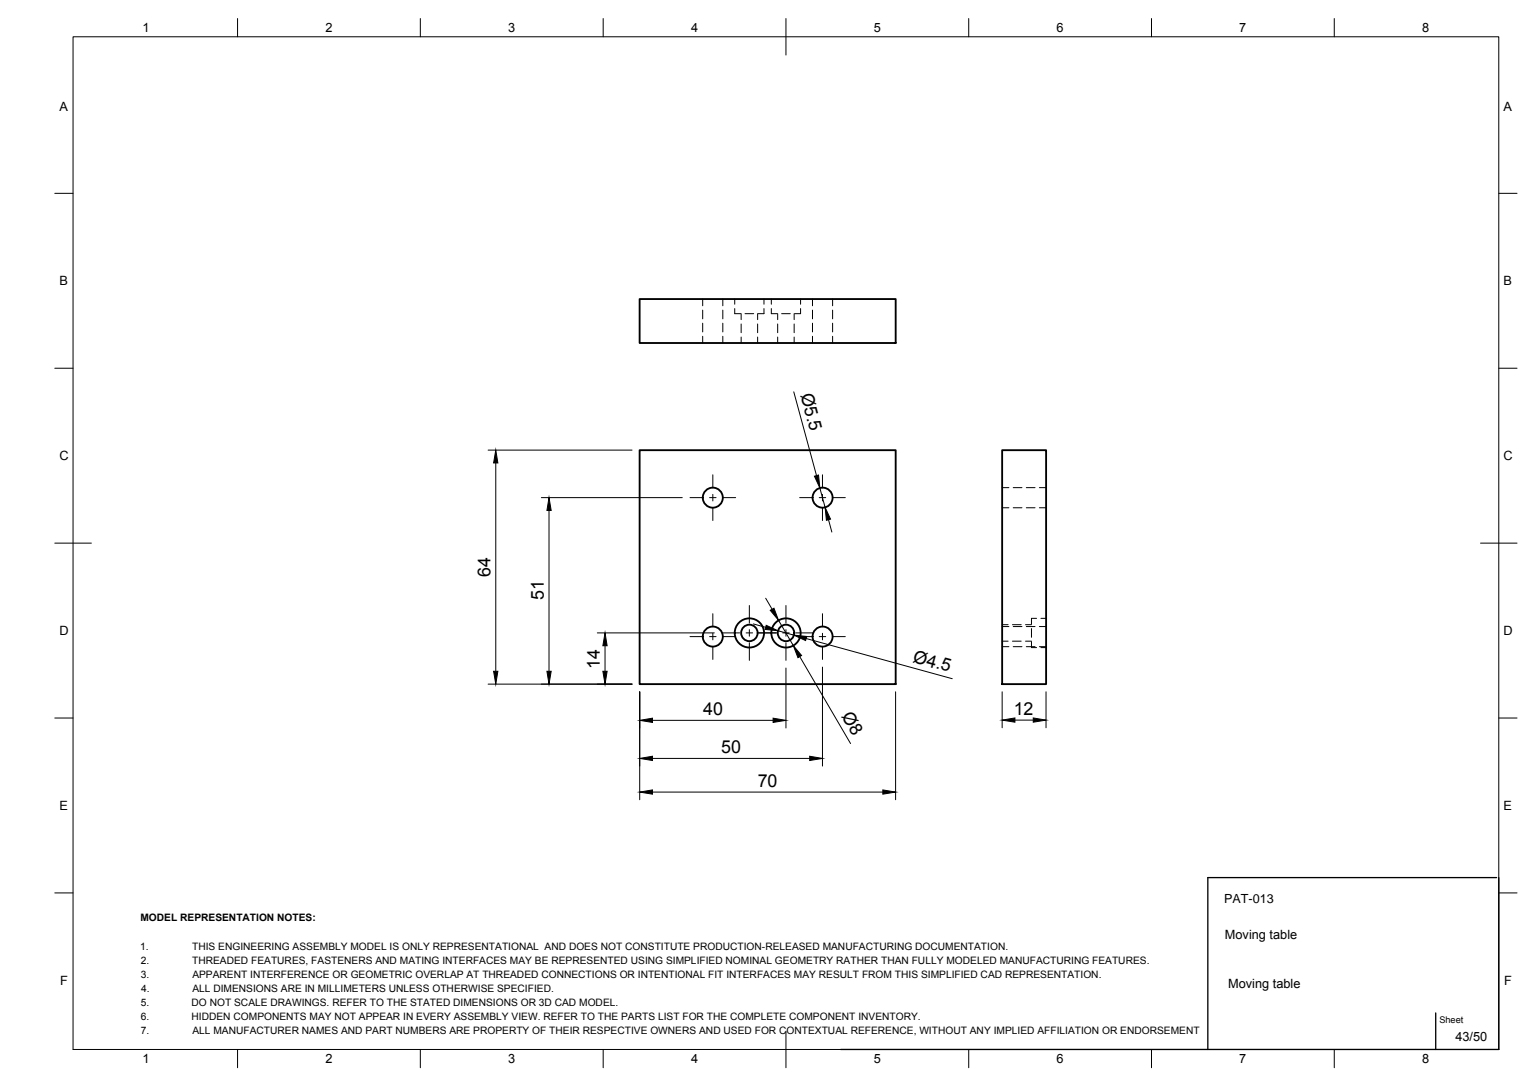
ISO-10303-21;
HEADER;
/* Generated by software containing ST-Developer
 * from STEP Tools, Inc. (www.steptools.com) 
 */

FILE_DESCRIPTION(
/* description */ ('Belt-driven linear axis on 2020 extrusion'),
/* implementation_level */ '2;1');

FILE_NAME(
/* name */ 'Moving table.step',
/* time_stamp */ '2026-10-28T03:26:09-07:00',
/* author */ (''),
/* organization */ (''),
/* preprocessor_version */ 'ST-DEVELOPER v20.2',
/* originating_system */ 'Autodesk Translation Framework v15.17.0.0',
/* authorisation */ '');

FILE_SCHEMA (('AUTOMOTIVE_DESIGN { 1 0 10303 214 3 1 1 }'));
ENDSEC;

DATA;
#10=MECHANICAL_DESIGN_GEOMETRIC_PRESENTATION_REPRESENTATION('',(#656),#20096);
#554=SHAPE_REPRESENTATION_RELATIONSHIP('SRR','None',#20354,#600);
#600=ADVANCED_BREP_SHAPE_REPRESENTATION('',(#711),#20085);
#656=STYLED_ITEM('',(#20643),#711);
#711=MANIFOLD_SOLID_BREP('Body1',#10970);
#862=FACE_BOUND('',#2501,.T.);
#863=FACE_BOUND('',#2504,.T.);
#864=FACE_BOUND('',#2516,.T.);
#865=FACE_BOUND('',#2517,.T.);
#866=FACE_BOUND('',#2518,.T.);
#867=FACE_BOUND('',#2519,.T.);
#868=FACE_BOUND('',#2520,.T.);
#869=FACE_BOUND('',#2521,.T.);
#870=FACE_BOUND('',#2523,.T.);
#871=FACE_BOUND('',#2524,.T.);
#872=FACE_BOUND('',#2525,.T.);
#873=FACE_BOUND('',#2526,.T.);
#874=FACE_BOUND('',#2527,.T.);
#875=FACE_BOUND('',#2528,.T.);
#1149=PLANE('',#12467);
#1150=PLANE('',#12472);
#1151=PLANE('',#12490);
#1152=PLANE('',#12491);
#1153=PLANE('',#12492);
#1154=PLANE('',#12493);
#1155=PLANE('',#12494);
#1156=PLANE('',#12495);
#1733=FACE_OUTER_BOUND('',#2499,.T.);
#1734=FACE_OUTER_BOUND('',#2500,.T.);
#1735=FACE_OUTER_BOUND('',#2502,.T.);
#1736=FACE_OUTER_BOUND('',#2503,.T.);
#1737=FACE_OUTER_BOUND('',#2505,.T.);
#1738=FACE_OUTER_BOUND('',#2506,.T.);
#1739=FACE_OUTER_BOUND('',#2507,.T.);
#1740=FACE_OUTER_BOUND('',#2508,.T.);
#1741=FACE_OUTER_BOUND('',#2509,.T.);
#1742=FACE_OUTER_BOUND('',#2510,.T.);
#1743=FACE_OUTER_BOUND('',#2511,.T.);
#1744=FACE_OUTER_BOUND('',#2512,.T.);
#1745=FACE_OUTER_BOUND('',#2513,.T.);
#1746=FACE_OUTER_BOUND('',#2514,.T.);
#1747=FACE_OUTER_BOUND('',#2515,.T.);
#1748=FACE_OUTER_BOUND('',#2522,.T.);
#2499=EDGE_LOOP('',(#9453,#9454,#9455,#9456));
#2500=EDGE_LOOP('',(#9457));
#2501=EDGE_LOOP('',(#9458));
#2502=EDGE_LOOP('',(#9459,#9460,#9461,#9462));
#2503=EDGE_LOOP('',(#9463));
#2504=EDGE_LOOP('',(#9464));
#2505=EDGE_LOOP('',(#9465,#9466,#9467,#9468));
#2506=EDGE_LOOP('',(#9469,#9470,#9471,#9472));
#2507=EDGE_LOOP('',(#9473,#9474,#9475,#9476));
#2508=EDGE_LOOP('',(#9477,#9478,#9479,#9480));
#2509=EDGE_LOOP('',(#9481,#9482,#9483,#9484));
#2510=EDGE_LOOP('',(#9485,#9486,#9487,#9488));
#2511=EDGE_LOOP('',(#9489,#9490,#9491,#9492));
#2512=EDGE_LOOP('',(#9493,#9494,#9495,#9496));
#2513=EDGE_LOOP('',(#9497,#9498,#9499,#9500));
#2514=EDGE_LOOP('',(#9501,#9502,#9503,#9504));
#2515=EDGE_LOOP('',(#9505,#9506,#9507,#9508));
#2516=EDGE_LOOP('',(#9509));
#2517=EDGE_LOOP('',(#9510));
#2518=EDGE_LOOP('',(#9511));
#2519=EDGE_LOOP('',(#9512));
#2520=EDGE_LOOP('',(#9513));
#2521=EDGE_LOOP('',(#9514));
#2522=EDGE_LOOP('',(#9515,#9516,#9517,#9518));
#2523=EDGE_LOOP('',(#9519));
#2524=EDGE_LOOP('',(#9520));
#2525=EDGE_LOOP('',(#9521));
#2526=EDGE_LOOP('',(#9522));
#2527=EDGE_LOOP('',(#9523));
#2528=EDGE_LOOP('',(#9524));
#3282=LINE('',#19228,#4139);
#3283=LINE('',#19237,#4140);
#3284=LINE('',#19244,#4141);
#3285=LINE('',#19248,#4142);
#3286=LINE('',#19254,#4143);
#3287=LINE('',#19260,#4144);
#3288=LINE('',#19266,#4145);
#3289=LINE('',#19272,#4146);
#3290=LINE('',#19277,#4147);
#3291=LINE('',#19279,#4148);
#3292=LINE('',#19281,#4149);
#3293=LINE('',#19282,#4150);
#3294=LINE('',#19285,#4151);
#3295=LINE('',#19287,#4152);
#3296=LINE('',#19288,#4153);
#3297=LINE('',#19291,#4154);
#3298=LINE('',#19293,#4155);
#3299=LINE('',#19294,#4156);
#3300=LINE('',#19296,#4157);
#3301=LINE('',#19297,#4158);
#4139=VECTOR('',#15354,0.4);
#4140=VECTOR('',#15365,0.399999999999999);
#4141=VECTOR('',#15374,0.225);
#4142=VECTOR('',#15379,0.225000000000001);
#4143=VECTOR('',#15386,0.274999999999999);
#4144=VECTOR('',#15393,0.275);
#4145=VECTOR('',#15400,0.275);
#4146=VECTOR('',#15407,0.274999999999999);
#4147=VECTOR('',#15412,1.);
#4148=VECTOR('',#15413,1.);
#4149=VECTOR('',#15414,1.);
#4150=VECTOR('',#15415,1.);
#4151=VECTOR('',#15418,1.);
#4152=VECTOR('',#15419,1.);
#4153=VECTOR('',#15420,1.);
#4154=VECTOR('',#15423,1.);
#4155=VECTOR('',#15424,1.);
#4156=VECTOR('',#15425,1.);
#4157=VECTOR('',#15428,1.);
#4158=VECTOR('',#15429,1.);
#4820=CIRCLE('',#12465,0.4);
#4821=CIRCLE('',#12466,0.4);
#4822=CIRCLE('',#12468,0.225);
#4823=CIRCLE('',#12470,0.399999999999999);
#4824=CIRCLE('',#12471,0.399999999999999);
#4825=CIRCLE('',#12473,0.225000000000001);
#4826=CIRCLE('',#12475,0.225);
#4827=CIRCLE('',#12477,0.225000000000001);
#4828=CIRCLE('',#12479,0.274999999999999);
#4829=CIRCLE('',#12480,0.274999999999999);
#4830=CIRCLE('',#12482,0.275);
#4831=CIRCLE('',#12483,0.275);
#4832=CIRCLE('',#12485,0.275);
#4833=CIRCLE('',#12486,0.275);
#4834=CIRCLE('',#12488,0.274999999999999);
#4835=CIRCLE('',#12489,0.274999999999999);
#5637=VERTEX_POINT('',#19225);
#5638=VERTEX_POINT('',#19227);
#5639=VERTEX_POINT('',#19231);
#5640=VERTEX_POINT('',#19234);
#5641=VERTEX_POINT('',#19236);
#5642=VERTEX_POINT('',#19240);
#5643=VERTEX_POINT('',#19243);
#5644=VERTEX_POINT('',#19247);
#5645=VERTEX_POINT('',#19251);
#5646=VERTEX_POINT('',#19253);
#5647=VERTEX_POINT('',#19257);
#5648=VERTEX_POINT('',#19259);
#5649=VERTEX_POINT('',#19263);
#5650=VERTEX_POINT('',#19265);
#5651=VERTEX_POINT('',#19269);
#5652=VERTEX_POINT('',#19271);
#5653=VERTEX_POINT('',#19275);
#5654=VERTEX_POINT('',#19276);
#5655=VERTEX_POINT('',#19278);
#5656=VERTEX_POINT('',#19280);
#5657=VERTEX_POINT('',#19284);
#5658=VERTEX_POINT('',#19286);
#5659=VERTEX_POINT('',#19290);
#5660=VERTEX_POINT('',#19292);
#6941=EDGE_CURVE('',#5637,#5637,#4820,.T.);
#6942=EDGE_CURVE('',#5637,#5638,#3282,.T.);
#6943=EDGE_CURVE('',#5638,#5638,#4821,.T.);
#6944=EDGE_CURVE('',#5639,#5639,#4822,.T.);
#6945=EDGE_CURVE('',#5640,#5640,#4823,.T.);
#6946=EDGE_CURVE('',#5640,#5641,#3283,.T.);
#6947=EDGE_CURVE('',#5641,#5641,#4824,.T.);
#6948=EDGE_CURVE('',#5642,#5642,#4825,.T.);
#6949=EDGE_CURVE('',#5639,#5643,#3284,.T.);
#6950=EDGE_CURVE('',#5643,#5643,#4826,.T.);
#6951=EDGE_CURVE('',#5642,#5644,#3285,.T.);
#6952=EDGE_CURVE('',#5644,#5644,#4827,.T.);
#6953=EDGE_CURVE('',#5645,#5645,#4828,.T.);
#6954=EDGE_CURVE('',#5645,#5646,#3286,.T.);
#6955=EDGE_CURVE('',#5646,#5646,#4829,.T.);
#6956=EDGE_CURVE('',#5647,#5647,#4830,.T.);
#6957=EDGE_CURVE('',#5647,#5648,#3287,.T.);
#6958=EDGE_CURVE('',#5648,#5648,#4831,.T.);
#6959=EDGE_CURVE('',#5649,#5649,#4832,.T.);
#6960=EDGE_CURVE('',#5649,#5650,#3288,.T.);
#6961=EDGE_CURVE('',#5650,#5650,#4833,.T.);
#6962=EDGE_CURVE('',#5651,#5651,#4834,.T.);
#6963=EDGE_CURVE('',#5651,#5652,#3289,.T.);
#6964=EDGE_CURVE('',#5652,#5652,#4835,.T.);
#6965=EDGE_CURVE('',#5653,#5654,#3290,.T.);
#6966=EDGE_CURVE('',#5654,#5655,#3291,.T.);
#6967=EDGE_CURVE('',#5656,#5655,#3292,.T.);
#6968=EDGE_CURVE('',#5653,#5656,#3293,.T.);
#6969=EDGE_CURVE('',#5657,#5653,#3294,.T.);
#6970=EDGE_CURVE('',#5658,#5656,#3295,.T.);
#6971=EDGE_CURVE('',#5657,#5658,#3296,.T.);
#6972=EDGE_CURVE('',#5659,#5657,#3297,.T.);
#6973=EDGE_CURVE('',#5660,#5658,#3298,.T.);
#6974=EDGE_CURVE('',#5659,#5660,#3299,.T.);
#6975=EDGE_CURVE('',#5654,#5659,#3300,.T.);
#6976=EDGE_CURVE('',#5655,#5660,#3301,.T.);
#9453=ORIENTED_EDGE('',*,*,#6941,.F.);
#9454=ORIENTED_EDGE('',*,*,#6942,.T.);
#9455=ORIENTED_EDGE('',*,*,#6943,.T.);
#9456=ORIENTED_EDGE('',*,*,#6942,.F.);
#9457=ORIENTED_EDGE('',*,*,#6943,.F.);
#9458=ORIENTED_EDGE('',*,*,#6944,.F.);
#9459=ORIENTED_EDGE('',*,*,#6945,.F.);
#9460=ORIENTED_EDGE('',*,*,#6946,.T.);
#9461=ORIENTED_EDGE('',*,*,#6947,.T.);
#9462=ORIENTED_EDGE('',*,*,#6946,.F.);
#9463=ORIENTED_EDGE('',*,*,#6947,.F.);
#9464=ORIENTED_EDGE('',*,*,#6948,.F.);
#9465=ORIENTED_EDGE('',*,*,#6944,.T.);
#9466=ORIENTED_EDGE('',*,*,#6949,.T.);
#9467=ORIENTED_EDGE('',*,*,#6950,.F.);
#9468=ORIENTED_EDGE('',*,*,#6949,.F.);
#9469=ORIENTED_EDGE('',*,*,#6948,.T.);
#9470=ORIENTED_EDGE('',*,*,#6951,.T.);
#9471=ORIENTED_EDGE('',*,*,#6952,.F.);
#9472=ORIENTED_EDGE('',*,*,#6951,.F.);
#9473=ORIENTED_EDGE('',*,*,#6953,.F.);
#9474=ORIENTED_EDGE('',*,*,#6954,.T.);
#9475=ORIENTED_EDGE('',*,*,#6955,.F.);
#9476=ORIENTED_EDGE('',*,*,#6954,.F.);
#9477=ORIENTED_EDGE('',*,*,#6956,.F.);
#9478=ORIENTED_EDGE('',*,*,#6957,.T.);
#9479=ORIENTED_EDGE('',*,*,#6958,.F.);
#9480=ORIENTED_EDGE('',*,*,#6957,.F.);
#9481=ORIENTED_EDGE('',*,*,#6959,.F.);
#9482=ORIENTED_EDGE('',*,*,#6960,.T.);
#9483=ORIENTED_EDGE('',*,*,#6961,.F.);
#9484=ORIENTED_EDGE('',*,*,#6960,.F.);
#9485=ORIENTED_EDGE('',*,*,#6962,.F.);
#9486=ORIENTED_EDGE('',*,*,#6963,.T.);
#9487=ORIENTED_EDGE('',*,*,#6964,.F.);
#9488=ORIENTED_EDGE('',*,*,#6963,.F.);
#9489=ORIENTED_EDGE('',*,*,#6965,.T.);
#9490=ORIENTED_EDGE('',*,*,#6966,.T.);
#9491=ORIENTED_EDGE('',*,*,#6967,.F.);
#9492=ORIENTED_EDGE('',*,*,#6968,.F.);
#9493=ORIENTED_EDGE('',*,*,#6969,.T.);
#9494=ORIENTED_EDGE('',*,*,#6968,.T.);
#9495=ORIENTED_EDGE('',*,*,#6970,.F.);
#9496=ORIENTED_EDGE('',*,*,#6971,.F.);
#9497=ORIENTED_EDGE('',*,*,#6972,.T.);
#9498=ORIENTED_EDGE('',*,*,#6971,.T.);
#9499=ORIENTED_EDGE('',*,*,#6973,.F.);
#9500=ORIENTED_EDGE('',*,*,#6974,.F.);
#9501=ORIENTED_EDGE('',*,*,#6975,.T.);
#9502=ORIENTED_EDGE('',*,*,#6974,.T.);
#9503=ORIENTED_EDGE('',*,*,#6976,.F.);
#9504=ORIENTED_EDGE('',*,*,#6966,.F.);
#9505=ORIENTED_EDGE('',*,*,#6976,.T.);
#9506=ORIENTED_EDGE('',*,*,#6973,.T.);
#9507=ORIENTED_EDGE('',*,*,#6970,.T.);
#9508=ORIENTED_EDGE('',*,*,#6967,.T.);
#9509=ORIENTED_EDGE('',*,*,#6950,.T.);
#9510=ORIENTED_EDGE('',*,*,#6952,.T.);
#9511=ORIENTED_EDGE('',*,*,#6955,.T.);
#9512=ORIENTED_EDGE('',*,*,#6958,.T.);
#9513=ORIENTED_EDGE('',*,*,#6961,.T.);
#9514=ORIENTED_EDGE('',*,*,#6964,.T.);
#9515=ORIENTED_EDGE('',*,*,#6975,.F.);
#9516=ORIENTED_EDGE('',*,*,#6965,.F.);
#9517=ORIENTED_EDGE('',*,*,#6969,.F.);
#9518=ORIENTED_EDGE('',*,*,#6972,.F.);
#9519=ORIENTED_EDGE('',*,*,#6962,.T.);
#9520=ORIENTED_EDGE('',*,*,#6959,.T.);
#9521=ORIENTED_EDGE('',*,*,#6956,.T.);
#9522=ORIENTED_EDGE('',*,*,#6953,.T.);
#9523=ORIENTED_EDGE('',*,*,#6945,.T.);
#9524=ORIENTED_EDGE('',*,*,#6941,.T.);
#10275=CYLINDRICAL_SURFACE('',#12464,0.4);
#10276=CYLINDRICAL_SURFACE('',#12469,0.399999999999999);
#10277=CYLINDRICAL_SURFACE('',#12474,0.225);
#10278=CYLINDRICAL_SURFACE('',#12476,0.225000000000001);
#10279=CYLINDRICAL_SURFACE('',#12478,0.274999999999999);
#10280=CYLINDRICAL_SURFACE('',#12481,0.275);
#10281=CYLINDRICAL_SURFACE('',#12484,0.275);
#10282=CYLINDRICAL_SURFACE('',#12487,0.274999999999999);
#10784=ADVANCED_FACE('',(#1733),#10275,.F.);
#10785=ADVANCED_FACE('',(#1734,#862),#1149,.F.);
#10786=ADVANCED_FACE('',(#1735),#10276,.F.);
#10787=ADVANCED_FACE('',(#1736,#863),#1150,.F.);
#10788=ADVANCED_FACE('',(#1737),#10277,.F.);
#10789=ADVANCED_FACE('',(#1738),#10278,.F.);
#10790=ADVANCED_FACE('',(#1739),#10279,.F.);
#10791=ADVANCED_FACE('',(#1740),#10280,.F.);
#10792=ADVANCED_FACE('',(#1741),#10281,.F.);
#10793=ADVANCED_FACE('',(#1742),#10282,.F.);
#10794=ADVANCED_FACE('',(#1743),#1151,.T.);
#10795=ADVANCED_FACE('',(#1744),#1152,.T.);
#10796=ADVANCED_FACE('',(#1745),#1153,.T.);
#10797=ADVANCED_FACE('',(#1746),#1154,.T.);
#10798=ADVANCED_FACE('',(#1747,#864,#865,#866,#867,#868,#869),#1155,.T.);
#10799=ADVANCED_FACE('',(#1748,#870,#871,#872,#873,#874,#875),#1156,.F.);
#10970=CLOSED_SHELL('',(#10784,#10785,#10786,#10787,#10788,#10789,#10790,
#10791,#10792,#10793,#10794,#10795,#10796,#10797,#10798,#10799));
#12463=AXIS2_PLACEMENT_3D('',#19223,#15348,#15349);
#12464=AXIS2_PLACEMENT_3D('',#19224,#15350,#15351);
#12465=AXIS2_PLACEMENT_3D('',#19226,#15352,#15353);
#12466=AXIS2_PLACEMENT_3D('',#19229,#15355,#15356);
#12467=AXIS2_PLACEMENT_3D('',#19230,#15357,#15358);
#12468=AXIS2_PLACEMENT_3D('',#19232,#15359,#15360);
#12469=AXIS2_PLACEMENT_3D('',#19233,#15361,#15362);
#12470=AXIS2_PLACEMENT_3D('',#19235,#15363,#15364);
#12471=AXIS2_PLACEMENT_3D('',#19238,#15366,#15367);
#12472=AXIS2_PLACEMENT_3D('',#19239,#15368,#15369);
#12473=AXIS2_PLACEMENT_3D('',#19241,#15370,#15371);
#12474=AXIS2_PLACEMENT_3D('',#19242,#15372,#15373);
#12475=AXIS2_PLACEMENT_3D('',#19245,#15375,#15376);
#12476=AXIS2_PLACEMENT_3D('',#19246,#15377,#15378);
#12477=AXIS2_PLACEMENT_3D('',#19249,#15380,#15381);
#12478=AXIS2_PLACEMENT_3D('',#19250,#15382,#15383);
#12479=AXIS2_PLACEMENT_3D('',#19252,#15384,#15385);
#12480=AXIS2_PLACEMENT_3D('',#19255,#15387,#15388);
#12481=AXIS2_PLACEMENT_3D('',#19256,#15389,#15390);
#12482=AXIS2_PLACEMENT_3D('',#19258,#15391,#15392);
#12483=AXIS2_PLACEMENT_3D('',#19261,#15394,#15395);
#12484=AXIS2_PLACEMENT_3D('',#19262,#15396,#15397);
#12485=AXIS2_PLACEMENT_3D('',#19264,#15398,#15399);
#12486=AXIS2_PLACEMENT_3D('',#19267,#15401,#15402);
#12487=AXIS2_PLACEMENT_3D('',#19268,#15403,#15404);
#12488=AXIS2_PLACEMENT_3D('',#19270,#15405,#15406);
#12489=AXIS2_PLACEMENT_3D('',#19273,#15408,#15409);
#12490=AXIS2_PLACEMENT_3D('',#19274,#15410,#15411);
#12491=AXIS2_PLACEMENT_3D('',#19283,#15416,#15417);
#12492=AXIS2_PLACEMENT_3D('',#19289,#15421,#15422);
#12493=AXIS2_PLACEMENT_3D('',#19295,#15426,#15427);
#12494=AXIS2_PLACEMENT_3D('',#19298,#15430,#15431);
#12495=AXIS2_PLACEMENT_3D('',#19299,#15432,#15433);
#15348=DIRECTION('axis',(0.,0.,1.));
#15349=DIRECTION('refdir',(1.,0.,0.));
#15350=DIRECTION('center_axis',(0.,0.,1.));
#15351=DIRECTION('ref_axis',(1.,0.,0.));
#15352=DIRECTION('center_axis',(0.,0.,1.));
#15353=DIRECTION('ref_axis',(1.,0.,0.));
#15354=DIRECTION('',(0.,0.,1.));
#15355=DIRECTION('center_axis',(0.,0.,1.));
#15356=DIRECTION('ref_axis',(1.,0.,0.));
#15357=DIRECTION('center_axis',(0.,0.,1.));
#15358=DIRECTION('ref_axis',(1.,0.,0.));
#15359=DIRECTION('center_axis',(0.,0.,-1.));
#15360=DIRECTION('ref_axis',(1.,0.,0.));
#15361=DIRECTION('center_axis',(0.,0.,1.));
#15362=DIRECTION('ref_axis',(1.,0.,0.));
#15363=DIRECTION('center_axis',(0.,0.,1.));
#15364=DIRECTION('ref_axis',(1.,0.,0.));
#15365=DIRECTION('',(0.,0.,1.));
#15366=DIRECTION('center_axis',(0.,0.,1.));
#15367=DIRECTION('ref_axis',(1.,0.,0.));
#15368=DIRECTION('center_axis',(0.,0.,1.));
#15369=DIRECTION('ref_axis',(1.,0.,0.));
#15370=DIRECTION('center_axis',(0.,0.,-1.));
#15371=DIRECTION('ref_axis',(1.,0.,0.));
#15372=DIRECTION('center_axis',(0.,0.,1.));
#15373=DIRECTION('ref_axis',(1.,0.,0.));
#15374=DIRECTION('',(0.,0.,1.));
#15375=DIRECTION('center_axis',(0.,0.,-1.));
#15376=DIRECTION('ref_axis',(1.,0.,0.));
#15377=DIRECTION('center_axis',(0.,0.,1.));
#15378=DIRECTION('ref_axis',(1.,0.,0.));
#15379=DIRECTION('',(0.,0.,1.));
#15380=DIRECTION('center_axis',(0.,0.,-1.));
#15381=DIRECTION('ref_axis',(1.,0.,0.));
#15382=DIRECTION('center_axis',(0.,0.,1.));
#15383=DIRECTION('ref_axis',(1.,0.,0.));
#15384=DIRECTION('center_axis',(0.,0.,1.));
#15385=DIRECTION('ref_axis',(1.,0.,0.));
#15386=DIRECTION('',(0.,0.,1.));
#15387=DIRECTION('center_axis',(0.,0.,-1.));
#15388=DIRECTION('ref_axis',(1.,0.,0.));
#15389=DIRECTION('center_axis',(0.,0.,1.));
#15390=DIRECTION('ref_axis',(1.,0.,0.));
#15391=DIRECTION('center_axis',(0.,0.,1.));
#15392=DIRECTION('ref_axis',(1.,0.,0.));
#15393=DIRECTION('',(0.,0.,1.));
#15394=DIRECTION('center_axis',(0.,0.,-1.));
#15395=DIRECTION('ref_axis',(1.,0.,0.));
#15396=DIRECTION('center_axis',(0.,0.,1.));
#15397=DIRECTION('ref_axis',(1.,0.,0.));
#15398=DIRECTION('center_axis',(0.,0.,1.));
#15399=DIRECTION('ref_axis',(1.,0.,0.));
#15400=DIRECTION('',(0.,0.,1.));
#15401=DIRECTION('center_axis',(0.,0.,-1.));
#15402=DIRECTION('ref_axis',(1.,0.,0.));
#15403=DIRECTION('center_axis',(0.,0.,1.));
#15404=DIRECTION('ref_axis',(1.,0.,0.));
#15405=DIRECTION('center_axis',(0.,0.,1.));
#15406=DIRECTION('ref_axis',(1.,0.,0.));
#15407=DIRECTION('',(0.,0.,1.));
#15408=DIRECTION('center_axis',(0.,0.,-1.));
#15409=DIRECTION('ref_axis',(1.,0.,0.));
#15410=DIRECTION('center_axis',(0.,1.,0.));
#15411=DIRECTION('ref_axis',(-1.,0.,0.));
#15412=DIRECTION('',(-1.,0.,0.));
#15413=DIRECTION('',(0.,0.,1.));
#15414=DIRECTION('',(-1.,0.,0.));
#15415=DIRECTION('',(0.,0.,1.));
#15416=DIRECTION('center_axis',(1.,0.,0.));
#15417=DIRECTION('ref_axis',(0.,1.,0.));
#15418=DIRECTION('',(0.,1.,0.));
#15419=DIRECTION('',(0.,1.,0.));
#15420=DIRECTION('',(0.,0.,1.));
#15421=DIRECTION('center_axis',(0.,-1.,0.));
#15422=DIRECTION('ref_axis',(1.,0.,0.));
#15423=DIRECTION('',(1.,0.,0.));
#15424=DIRECTION('',(1.,0.,0.));
#15425=DIRECTION('',(0.,0.,1.));
#15426=DIRECTION('center_axis',(-1.,0.,0.));
#15427=DIRECTION('ref_axis',(0.,-1.,0.));
#15428=DIRECTION('',(0.,-1.,0.));
#15429=DIRECTION('',(0.,-1.,0.));
#15430=DIRECTION('center_axis',(0.,0.,1.));
#15431=DIRECTION('ref_axis',(1.,0.,0.));
#15432=DIRECTION('center_axis',(0.,0.,1.));
#15433=DIRECTION('ref_axis',(1.,0.,0.));
#19223=CARTESIAN_POINT('',(0.,0.,0.));
#19224=CARTESIAN_POINT('Origin',(15.5,-1.8,2.3));
#19225=CARTESIAN_POINT('',(15.1,-1.8,2.4));
#19226=CARTESIAN_POINT('Origin',(15.5,-1.8,2.4));
#19227=CARTESIAN_POINT('',(15.1,-1.8,2.8));
#19228=CARTESIAN_POINT('',(15.1,-1.8,2.3));
#19229=CARTESIAN_POINT('Origin',(15.5,-1.8,2.8));
#19230=CARTESIAN_POINT('Origin',(15.5,-1.8,2.8));
#19231=CARTESIAN_POINT('',(15.275,-1.8,2.8));
#19232=CARTESIAN_POINT('Origin',(15.5,-1.8,2.8));
#19233=CARTESIAN_POINT('Origin',(16.5,-1.8,2.3));
#19234=CARTESIAN_POINT('',(16.1,-1.8,2.4));
#19235=CARTESIAN_POINT('Origin',(16.5,-1.8,2.4));
#19236=CARTESIAN_POINT('',(16.1,-1.8,2.8));
#19237=CARTESIAN_POINT('',(16.1,-1.8,2.3));
#19238=CARTESIAN_POINT('Origin',(16.5,-1.8,2.8));
#19239=CARTESIAN_POINT('Origin',(16.5,-1.8,2.8));
#19240=CARTESIAN_POINT('',(16.275,-1.8,2.8));
#19241=CARTESIAN_POINT('Origin',(16.5,-1.8,2.8));
#19242=CARTESIAN_POINT('Origin',(15.5,-1.8,2.3));
#19243=CARTESIAN_POINT('',(15.275,-1.8,3.6));
#19244=CARTESIAN_POINT('',(15.275,-1.8,2.3));
#19245=CARTESIAN_POINT('Origin',(15.5,-1.8,3.6));
#19246=CARTESIAN_POINT('Origin',(16.5,-1.8,2.3));
#19247=CARTESIAN_POINT('',(16.275,-1.8,3.6));
#19248=CARTESIAN_POINT('',(16.275,-1.8,2.3));
#19249=CARTESIAN_POINT('Origin',(16.5,-1.8,3.6));
#19250=CARTESIAN_POINT('Origin',(17.5,-1.9,2.3));
#19251=CARTESIAN_POINT('',(17.225,-1.9,2.4));
#19252=CARTESIAN_POINT('Origin',(17.5,-1.9,2.4));
#19253=CARTESIAN_POINT('',(17.225,-1.9,3.6));
#19254=CARTESIAN_POINT('',(17.225,-1.9,2.3));
#19255=CARTESIAN_POINT('Origin',(17.5,-1.9,3.6));
#19256=CARTESIAN_POINT('Origin',(14.5,1.9,2.3));
#19257=CARTESIAN_POINT('',(14.225,1.9,2.4));
#19258=CARTESIAN_POINT('Origin',(14.5,1.9,2.4));
#19259=CARTESIAN_POINT('',(14.225,1.9,3.6));
#19260=CARTESIAN_POINT('',(14.225,1.9,2.3));
#19261=CARTESIAN_POINT('Origin',(14.5,1.9,3.6));
#19262=CARTESIAN_POINT('Origin',(14.5,-1.9,2.3));
#19263=CARTESIAN_POINT('',(14.225,-1.9,2.4));
#19264=CARTESIAN_POINT('Origin',(14.5,-1.9,2.4));
#19265=CARTESIAN_POINT('',(14.225,-1.9,3.6));
#19266=CARTESIAN_POINT('',(14.225,-1.9,2.3));
#19267=CARTESIAN_POINT('Origin',(14.5,-1.9,3.6));
#19268=CARTESIAN_POINT('Origin',(17.5,1.9,2.3));
#19269=CARTESIAN_POINT('',(17.225,1.9,2.4));
#19270=CARTESIAN_POINT('Origin',(17.5,1.9,2.4));
#19271=CARTESIAN_POINT('',(17.225,1.9,3.6));
#19272=CARTESIAN_POINT('',(17.225,1.9,2.3));
#19273=CARTESIAN_POINT('Origin',(17.5,1.9,3.6));
#19274=CARTESIAN_POINT('Origin',(19.5,3.2,2.4));
#19275=CARTESIAN_POINT('',(19.5,3.2,2.4));
#19276=CARTESIAN_POINT('',(12.5,3.2,2.4));
#19277=CARTESIAN_POINT('',(19.5,3.2,2.4));
#19278=CARTESIAN_POINT('',(12.5,3.2,3.6));
#19279=CARTESIAN_POINT('',(12.5,3.2,2.4));
#19280=CARTESIAN_POINT('',(19.5,3.2,3.6));
#19281=CARTESIAN_POINT('',(19.5,3.2,3.6));
#19282=CARTESIAN_POINT('',(19.5,3.2,2.4));
#19283=CARTESIAN_POINT('Origin',(19.5,-3.2,2.4));
#19284=CARTESIAN_POINT('',(19.5,-3.2,2.4));
#19285=CARTESIAN_POINT('',(19.5,-3.2,2.4));
#19286=CARTESIAN_POINT('',(19.5,-3.2,3.6));
#19287=CARTESIAN_POINT('',(19.5,-3.2,3.6));
#19288=CARTESIAN_POINT('',(19.5,-3.2,2.4));
#19289=CARTESIAN_POINT('Origin',(12.5,-3.2,2.4));
#19290=CARTESIAN_POINT('',(12.5,-3.2,2.4));
#19291=CARTESIAN_POINT('',(12.5,-3.2,2.4));
#19292=CARTESIAN_POINT('',(12.5,-3.2,3.6));
#19293=CARTESIAN_POINT('',(12.5,-3.2,3.6));
#19294=CARTESIAN_POINT('',(12.5,-3.2,2.4));
#19295=CARTESIAN_POINT('Origin',(12.5,3.2,2.4));
#19296=CARTESIAN_POINT('',(12.5,3.2,2.4));
#19297=CARTESIAN_POINT('',(12.5,3.2,3.6));
#19298=CARTESIAN_POINT('Origin',(16.,0.,3.6));
#19299=CARTESIAN_POINT('Origin',(16.,0.,2.4));
#20031=UNCERTAINTY_MEASURE_WITH_UNIT(LENGTH_MEASURE(0.001),#20097,
'DISTANCE_ACCURACY_VALUE',
'Maximum model space distance between geometric entities at asserted c
onnectivities');
#20042=UNCERTAINTY_MEASURE_WITH_UNIT(LENGTH_MEASURE(0.001),#20097,
'DISTANCE_ACCURACY_VALUE',
'Maximum model space distance between geometric entities at asserted c
onnectivities');
#20085=(
GEOMETRIC_REPRESENTATION_CONTEXT(3)
GLOBAL_UNCERTAINTY_ASSIGNED_CONTEXT((#20031))
GLOBAL_UNIT_ASSIGNED_CONTEXT((#20097,#20099,#20100))
REPRESENTATION_CONTEXT('','3D')
);
#20096=(
GEOMETRIC_REPRESENTATION_CONTEXT(3)
GLOBAL_UNCERTAINTY_ASSIGNED_CONTEXT((#20042))
GLOBAL_UNIT_ASSIGNED_CONTEXT((#20097,#20099,#20100))
REPRESENTATION_CONTEXT('','3D')
);
#20097=(
LENGTH_UNIT()
NAMED_UNIT(*)
SI_UNIT(.CENTI.,.METRE.)
);
#20099=(
NAMED_UNIT(*)
PLANE_ANGLE_UNIT()
SI_UNIT($,.RADIAN.)
);
#20100=(
NAMED_UNIT(*)
SI_UNIT($,.STERADIAN.)
SOLID_ANGLE_UNIT()
);
#20143=SHAPE_DEFINITION_REPRESENTATION(#20201,#20354);
#20201=PRODUCT_DEFINITION_SHAPE('',$,#20408);
#20354=SHAPE_REPRESENTATION('',(#12463),#20085);
#20365=PRODUCT_DEFINITION_CONTEXT('part definition',#20526,'design');
#20408=PRODUCT_DEFINITION('Moving table','Moving table',#20461,#20365);
#20461=PRODUCT_DEFINITION_FORMATION('',$,#20570);
#20526=APPLICATION_CONTEXT(
'Core Data for Automotive Mechanical Design Process');
#20527=PRODUCT_CONTEXT('part definition',#20526,'mechanical');
#20570=PRODUCT('Moving table','Moving table','Moving table',(#20527));
#20637=COLOUR_RGB('Sky Blue',0.24,0.69,0.87);
#20638=FILL_AREA_STYLE_COLOUR('',#20637);
#20639=FILL_AREA_STYLE('',(#20638));
#20640=SURFACE_STYLE_FILL_AREA(#20639);
#20641=SURFACE_SIDE_STYLE('',(#20640));
#20642=SURFACE_STYLE_USAGE(.BOTH.,#20641);
#20643=PRESENTATION_STYLE_ASSIGNMENT((#20642));
ENDSEC;
END-ISO-10303-21;
